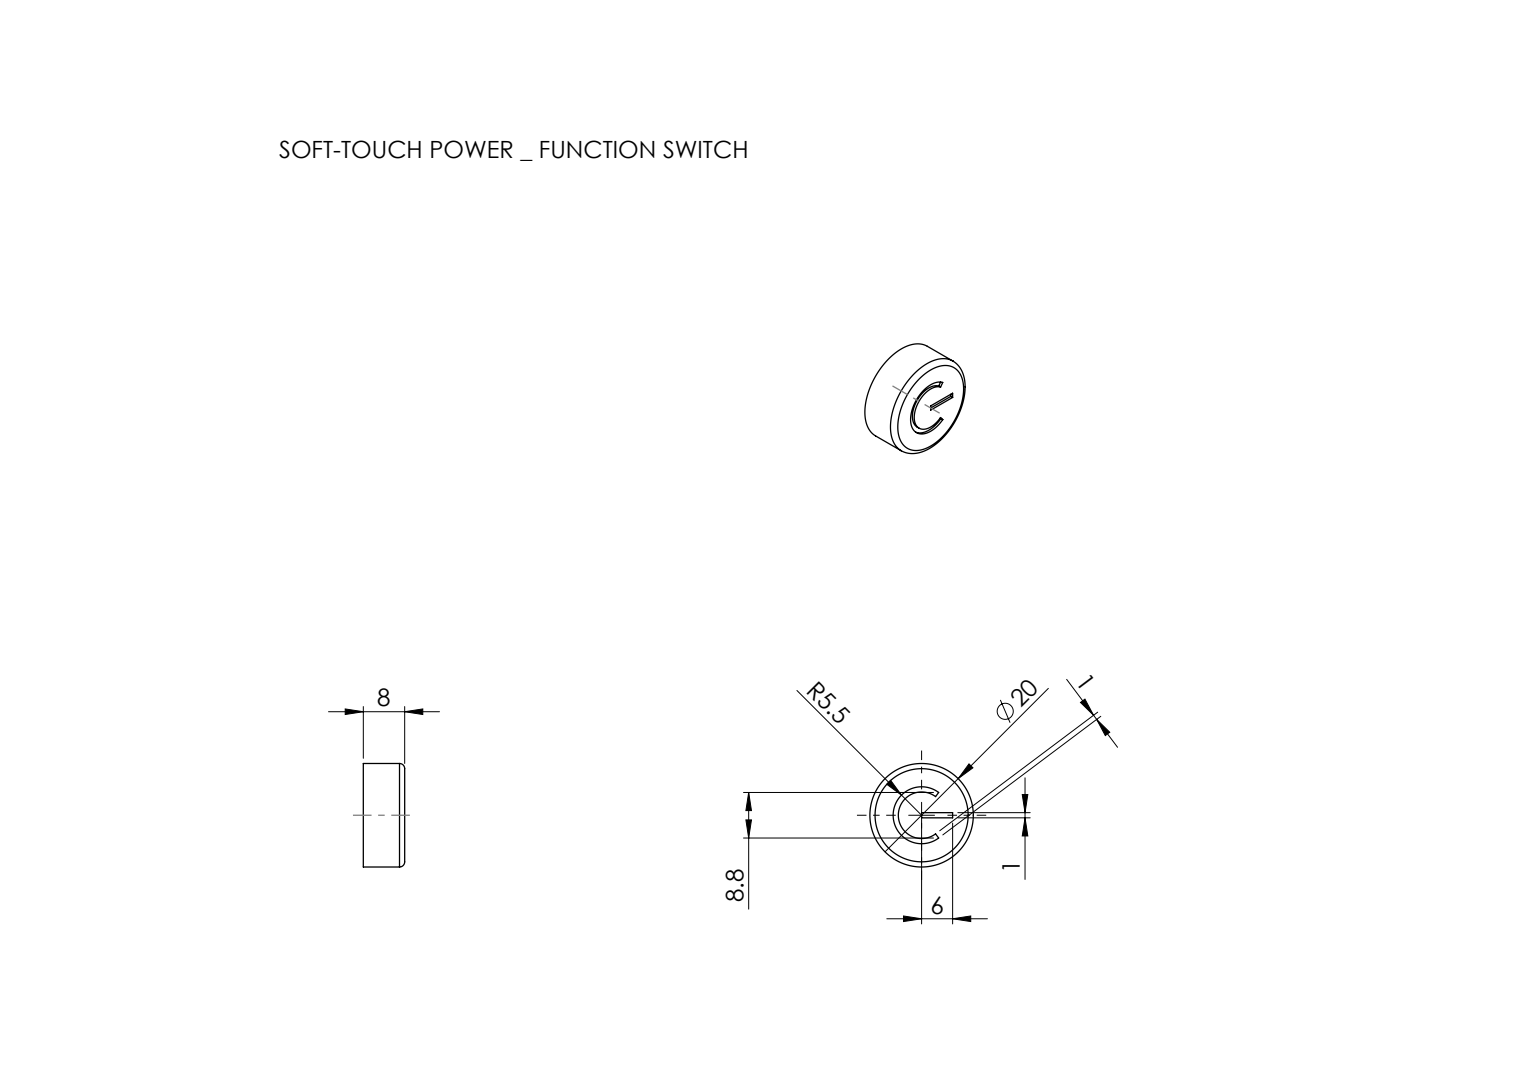
ISO-10303-21;
HEADER;
FILE_DESCRIPTION (('STEP AP214'),
    '1' );
FILE_NAME ('Soft-Touch Power _ Function Switch.step',
    '2026-10-08T15:02:10',
    ( '' ),
    ( '' ),
    'SwSTEP 2.0',
    'SolidWorks 2026',
    '' );
FILE_SCHEMA (( 'AUTOMOTIVE_DESIGN' ));
ENDSEC;

DATA;
#46=ORIENTED_EDGE ( 'NONE', *, *, #19993, .F. ) ;
#61=AXIS2_PLACEMENT_3D ( 'NONE', #8300, #8190, #21897 ) ;
#107=VECTOR ( 'NONE', #10777, 1000.000000000000000 ) ;
#129=CARTESIAN_POINT ( 'NONE',  ( 26.00000000000000000, -0.5000000000000000000, 0.000000000000000000 ) ) ;
#137=VERTEX_POINT ( 'NONE', #405 ) ;
#175=CARTESIAN_POINT ( 'NONE',  ( 26.00000000000000000, 0.5000000000000000000, 0.000000000000000000 ) ) ;
#230=DIRECTION ( 'NONE',  ( 0.000000000000000000, -1.000000000000000000, 0.000000000000000000 ) ) ;
#276=ORIENTED_EDGE ( 'NONE', *, *, #16709, .F. ) ;
#314=PRESENTATION_STYLE_ASSIGNMENT (( #17535 ) ) ;
#328=ORIENTED_EDGE ( 'NONE', *, *, #15715, .F. ) ;
#330=DIRECTION ( 'NONE',  ( 1.000000000000000000, 0.000000000000000000, 0.000000000000000000 ) ) ;
#379=FACE_OUTER_BOUND ( 'NONE', #20962, .T. ) ;
#386=EDGE_LOOP ( 'NONE', ( #10513, #13863, #2222, #14894 ) ) ;
#390=CARTESIAN_POINT ( 'NONE',  ( 25.50000000000000000, -0.5000000000000000000, 0.000000000000000000 ) ) ;
#405=CARTESIAN_POINT ( 'NONE',  ( 25.50000000000000000, -4.400000000000000355, -3.299999999999998490 ) ) ;
#408=DIRECTION ( 'NONE',  ( 1.000000000000000000, 0.000000000000000000, 0.000000000000000000 ) ) ;
#530=SURFACE_SIDE_STYLE ('',( #12575 ) ) ;
#566=VERTEX_POINT ( 'NONE', #2846 ) ;
#664=DIRECTION ( 'NONE',  ( 0.000000000000000000, 0.000000000000000000, -1.000000000000000000 ) ) ;
#679=AXIS2_PLACEMENT_3D ( 'NONE', #6039, #12809, #19760 ) ;
#731=CARTESIAN_POINT ( 'NONE',  ( 25.50000000000000000, 0.5000000000000000000, 0.000000000000000000 ) ) ;
#746=ADVANCED_FACE ( 'NONE', ( #18285 ), #1172, .T. ) ;
#770=CARTESIAN_POINT ( 'NONE',  ( 26.00000000000000000, 1.371657349757716727E-13, 9.000000000000001776 ) ) ;
#777=ORIENTED_EDGE ( 'NONE', *, *, #1994, .F. ) ;
#858=CARTESIAN_POINT ( 'NONE',  ( 26.00000000000000000, -0.5000000000000000000, 0.000000000000000000 ) ) ;
#976=ORIENTED_EDGE ( 'NONE', *, *, #5207, .F. ) ;
#1068=ORIENTED_EDGE ( 'NONE', *, *, #14661, .F. ) ;
#1075=CARTESIAN_POINT ( 'NONE',  ( 24.99999999999999645, 1.360023205165816762E-13, 10.00000000000000000 ) ) ;
#1088=ORIENTED_EDGE ( 'NONE', *, *, #2868, .F. ) ;
#1172=PLANE ( 'NONE',  #9056 ) ;
#1223=AXIS2_PLACEMENT_3D ( 'NONE', #21571, #2886, #14628 ) ;
#1293=EDGE_LOOP ( 'NONE', ( #4845, #14996, #17881, #4341 ) ) ;
#1397=VECTOR ( 'NONE', #13022, 1000.000000000000000 ) ;
#1428=PLANE ( 'NONE',  #21312 ) ;
#1693=DIRECTION ( 'NONE',  ( -1.000000000000000000, -0.000000000000000000, -0.000000000000000000 ) ) ;
#1761=LINE ( 'NONE', #8635, #13730 ) ;
#1967=DIRECTION ( 'NONE',  ( 0.000000000000000000, 0.000000000000000000, -1.000000000000000000 ) ) ;
#1994=EDGE_CURVE ( 'NONE', #6655, #4083, #3238, .T. ) ;
#2005=CARTESIAN_POINT ( 'NONE',  ( 26.00000000000000000, 0.000000000000000000, 0.000000000000000000 ) ) ;
#2048=DIRECTION ( 'NONE',  ( 1.000000000000000000, -0.000000000000000000, -0.000000000000000000 ) ) ;
#2170=AXIS2_PLACEMENT_3D ( 'NONE', #8967, #408, #3883 ) ;
#2214=ORIENTED_EDGE ( 'NONE', *, *, #11959, .F. ) ;
#2222=ORIENTED_EDGE ( 'NONE', *, *, #12958, .T. ) ;
#2243=ORIENTED_EDGE ( 'NONE', *, *, #15304, .F. ) ;
#2273=VECTOR ( 'NONE', #17556, 1000.000000000000000 ) ;
#2275=CARTESIAN_POINT ( 'NONE',  ( 26.00000000000000000, -4.400000000000000355, -3.299999999999998934 ) ) ;
#2285=ORIENTED_EDGE ( 'NONE', *, *, #5420, .T. ) ;
#2293=CARTESIAN_POINT ( 'NONE',  ( 24.99999999999999645, 1.371045026358143178E-13, 9.000000000000001776 ) ) ;
#2298=ORIENTED_EDGE ( 'NONE', *, *, #5629, .F. ) ;
#2331=CIRCLE ( 'NONE', #18866, 9.000000000000001776 ) ;
#2426=DIRECTION ( 'NONE',  ( 1.000000000000000000, -0.000000000000000000, -0.000000000000000000 ) ) ;
#2448=DIRECTION ( 'NONE',  ( -1.000000000000000000, 0.000000000000000000, -0.000000000000000000 ) ) ;
#2510=DIRECTION ( 'NONE',  ( 0.000000000000000000, -1.000000000000000000, 0.000000000000000000 ) ) ;
#2548=LINE ( 'NONE', #18093, #1397 ) ;
#2555=FACE_OUTER_BOUND ( 'NONE', #14128, .T. ) ;
#2588=ORIENTED_EDGE ( 'NONE', *, *, #4728, .F. ) ;
#2656=ORIENTED_EDGE ( 'NONE', *, *, #14942, .F. ) ;
#2672=EDGE_CURVE ( 'NONE', #6212, #9522, #7164, .T. ) ;
#2707=DIRECTION ( 'NONE',  ( 1.000000000000000000, 0.000000000000000000, 0.000000000000000000 ) ) ;
#2782=ADVANCED_FACE ( 'NONE', ( #19982 ), #6262, .F. ) ;
#2846=CARTESIAN_POINT ( 'NONE',  ( 25.50000000000000000, 0.5000000000000000000, -6.000000000000000000 ) ) ;
#2868=EDGE_CURVE ( 'NONE', #6745, #4083, #2548, .T. ) ;
#2886=DIRECTION ( 'NONE',  ( -1.000000000000000000, -0.000000000000000000, -0.000000000000000000 ) ) ;
#2913=FACE_OUTER_BOUND ( 'NONE', #3821, .T. ) ;
#2958=AXIS2_PLACEMENT_3D ( 'NONE', #14735, #19446, #4033 ) ;
#2986=CARTESIAN_POINT ( 'NONE',  ( 26.00000000000000000, 1.360023205165816762E-13, 0.000000000000000000 ) ) ;
#2998=( LENGTH_UNIT ( ) NAMED_UNIT ( * ) SI_UNIT ( .MILLI., .METRE. ) );
#3082=ORIENTED_EDGE ( 'NONE', *, *, #8473, .T. ) ;
#3119=CARTESIAN_POINT ( 'NONE',  ( 18.00000000000000000, 1.372269673157290277E-13, -10.00000000000000000 ) ) ;
#3159=CYLINDRICAL_SURFACE ( 'NONE', #11262, 4.500000000000000888 ) ;
#3238=LINE ( 'NONE', #3467, #7997 ) ;
#3252=EDGE_CURVE ( 'NONE', #12810, #12003, #3901, .T. ) ;
#3274=EDGE_LOOP ( 'NONE', ( #3082, #777, #2298, #22194 ) ) ;
#3321=CARTESIAN_POINT ( 'NONE',  ( 26.00000000000000000, -3.600000000000001421, -2.699999999999999289 ) ) ;
#3351=AXIS2_PLACEMENT_3D ( 'NONE', #14118, #5542, #19272 ) ;
#3391=VERTEX_POINT ( 'NONE', #3321 ) ;
#3436=DIRECTION ( 'NONE',  ( -1.000000000000000000, -0.000000000000000000, -0.000000000000000000 ) ) ;
#3467=CARTESIAN_POINT ( 'NONE',  ( 25.50000000000000000, -0.5000000000000000000, -6.000000000000000000 ) ) ;
#3474=ADVANCED_FACE ( 'NONE', ( #12002 ), #15162, .T. ) ;
#3756=DIRECTION ( 'NONE',  ( 0.000000000000000000, 1.000000000000000000, -1.224646799147353207E-16 ) ) ;
#3821=EDGE_LOOP ( 'NONE', ( #17497, #17029, #20739, #5281 ) ) ;
#3883=DIRECTION ( 'NONE',  ( 0.000000000000000000, 0.000000000000000000, -1.000000000000000000 ) ) ;
#3897=FILL_AREA_STYLE_COLOUR ( '', #6324 ) ;
#3901=CIRCLE ( 'NONE', #17927, 10.00000000000000000 ) ;
#4011=ORIENTED_EDGE ( 'NONE', *, *, #12403, .T. ) ;
#4032=LINE ( 'NONE', #21029, #9543 ) ;
#4033=DIRECTION ( 'NONE',  ( 0.000000000000000000, 0.000000000000000000, -1.000000000000000000 ) ) ;
#4043=AXIS2_PLACEMENT_3D ( 'NONE', #13177, #18133, #21596 ) ;
#4083=VERTEX_POINT ( 'NONE', #12114 ) ;
#4109=AXIS2_PLACEMENT_3D ( 'NONE', #10961, #16243, #16035 ) ;
#4115=CARTESIAN_POINT ( 'NONE',  ( 25.50000000000000000, -3.600000000000001421, -2.699999999999999289 ) ) ;
#4132=AXIS2_PLACEMENT_3D ( 'NONE', #7100, #230, #17449 ) ;
#4218=ORIENTED_EDGE ( 'NONE', *, *, #14942, .T. ) ;
#4341=ORIENTED_EDGE ( 'NONE', *, *, #14266, .F. ) ;
#4546=PRODUCT_CONTEXT ( 'NONE', #7149, 'mechanical' ) ;
#4609=DIRECTION ( 'NONE',  ( 0.000000000000000000, -0.7999999999999997113, 0.6000000000000004219 ) ) ;
#4614=CARTESIAN_POINT ( 'NONE',  ( 25.50000000000000000, 0.000000000000000000, 0.000000000000000000 ) ) ;
#4682=PRODUCT_DEFINITION_CONTEXT ( 'detailed design', #12889, 'design' ) ;
#4693=LINE ( 'NONE', #175, #9110 ) ;
#4720=SHAPE_REPRESENTATION_RELATIONSHIP ( 'NONE' , 'NONE' ,  #9901, #5876 ) ;
#4728=EDGE_CURVE ( 'NONE', #10662, #7309, #14691, .T. ) ;
#4793=DIRECTION ( 'NONE',  ( 0.000000000000000000, 1.000000000000000000, 0.000000000000000000 ) ) ;
#4845=ORIENTED_EDGE ( 'NONE', *, *, #5629, .T. ) ;
#4908=LINE ( 'NONE', #15393, #12641 ) ;
#5047=VECTOR ( 'NONE', #12562, 1000.000000000000000 ) ;
#5067=ORIENTED_EDGE ( 'NONE', *, *, #21758, .T. ) ;
#5125=DIRECTION ( 'NONE',  ( 0.000000000000000000, 0.000000000000000000, -1.000000000000000000 ) ) ;
#5207=EDGE_CURVE ( 'NONE', #10297, #15308, #1761, .T. ) ;
#5218=DIRECTION ( 'NONE',  ( 0.000000000000000000, 1.000000000000000000, 0.000000000000000000 ) ) ;
#5251=DIRECTION ( 'NONE',  ( 1.000000000000000000, -0.000000000000000000, -0.000000000000000000 ) ) ;
#5281=ORIENTED_EDGE ( 'NONE', *, *, #11865, .T. ) ;
#5358=CARTESIAN_POINT ( 'NONE',  ( 25.50000000000000000, -3.600000000000001421, -2.699999999999999289 ) ) ;
#5406=ADVANCED_FACE ( 'NONE', ( #8529 ), #13700, .T. ) ;
#5420=EDGE_CURVE ( 'NONE', #3391, #9522, #4908, .T. ) ;
#5519=DIRECTION ( 'NONE',  ( 0.000000000000000000, 0.000000000000000000, 1.000000000000000000 ) ) ;
#5531=DIRECTION ( 'NONE',  ( 0.000000000000000000, 0.000000000000000000, -1.000000000000000000 ) ) ;
#5542=DIRECTION ( 'NONE',  ( 1.000000000000000000, 0.000000000000000000, 0.000000000000000000 ) ) ;
#5592=DIRECTION ( 'NONE',  ( 0.000000000000000000, -0.7999999999999999334, -0.5999999999999999778 ) ) ;
#5624=ORIENTED_EDGE ( 'NONE', *, *, #15873, .T. ) ;
#5626=ORIENTED_EDGE ( 'NONE', *, *, #11865, .F. ) ;
#5629=EDGE_CURVE ( 'NONE', #15933, #6655, #6832, .T. ) ;
#5683=CARTESIAN_POINT ( 'NONE',  ( 25.50000000000000000, -0.5000000000000000000, 0.000000000000000000 ) ) ;
#5684=AXIS2_PLACEMENT_3D ( 'NONE', #2986, #3436, #20194 ) ;
#5695=CARTESIAN_POINT ( 'NONE',  ( 26.00000000000000000, 0.5000000000000000000, -6.000000000000000000 ) ) ;
#5819=EDGE_LOOP ( 'NONE', ( #17403, #18927 ) ) ;
#5855=PLANE ( 'NONE',  #4043 ) ;
#5870=DIRECTION ( 'NONE',  ( 0.000000000000000000, -0.7999999999999997113, 0.6000000000000004219 ) ) ;
#5873=EDGE_CURVE ( 'NONE', #19507, #13805, #10857, .T. ) ;
#5876=ADVANCED_BREP_SHAPE_REPRESENTATION ( '', ( #6798, #6677 ), #16347 ) ;
#5979=EDGE_CURVE ( 'NONE', #15933, #10297, #7395, .T. ) ;
#6039=CARTESIAN_POINT ( 'NONE',  ( 25.50000000000000000, -0.5000000000000000000, 0.000000000000000000 ) ) ;
#6045=CARTESIAN_POINT ( 'NONE',  ( 25.50000000000000000, -0.5000000000000000000, 0.000000000000000000 ) ) ;
#6048=FILL_AREA_STYLE ('',( #13253 ) ) ;
#6055=DIRECTION ( 'NONE',  ( 1.000000000000000000, 0.000000000000000000, 0.000000000000000000 ) ) ;
#6096=ADVANCED_FACE ( 'NONE', ( #8051 ), #16161, .T. ) ;
#6104=ADVANCED_FACE ( 'NONE', ( #12781 ), #21530, .T. ) ;
#6120=CARTESIAN_POINT ( 'NONE',  ( 26.00000000000000000, 4.399999999999999467, -3.300000000000000266 ) ) ;
#6212=VERTEX_POINT ( 'NONE', #6120 ) ;
#6262=PLANE ( 'NONE',  #679 ) ;
#6269=FACE_BOUND ( 'NONE', #11468, .T. ) ;
#6272=( NAMED_UNIT ( * ) SI_UNIT ( $, .STERADIAN. ) SOLID_ANGLE_UNIT ( ) );
#6296=AXIS2_PLACEMENT_3D ( 'NONE', #11354, #6055, #13153 ) ;
#6303=FACE_OUTER_BOUND ( 'NONE', #5819, .T. ) ;
#6324=COLOUR_RGB ( '', 0.09019608, 0.27058824, 0.51372549) ;
#6428=PRODUCT_DEFINITION ( 'UNKNOWN', '', #10679, #4682 ) ;
#6436=ORIENTED_EDGE ( 'NONE', *, *, #20861, .T. ) ;
#6606=DIRECTION ( 'NONE',  ( 0.000000000000000000, 0.000000000000000000, -1.000000000000000000 ) ) ;
#6617=CARTESIAN_POINT ( 'NONE',  ( 25.50000000000000000, -0.5000000000000000000, -6.000000000000000000 ) ) ;
#6655=VERTEX_POINT ( 'NONE', #6617 ) ;
#6662=DIRECTION ( 'NONE',  ( 1.000000000000000000, -0.000000000000000000, -0.000000000000000000 ) ) ;
#6677=AXIS2_PLACEMENT_3D ( 'NONE', #18028, #16226, #2707 ) ;
#6717=DIRECTION ( 'NONE',  ( 1.000000000000000000, 0.000000000000000000, 0.000000000000000000 ) ) ;
#6745=VERTEX_POINT ( 'NONE', #5695 ) ;
#6775=CARTESIAN_POINT ( 'NONE',  ( 25.50000000000000000, 0.000000000000000000, 0.000000000000000000 ) ) ;
#6798=MANIFOLD_SOLID_BREP ( 'Cut-Extrude-Thin1', #21569 ) ;
#6832=LINE ( 'NONE', #20535, #21975 ) ;
#6893=ORIENTED_EDGE ( 'NONE', *, *, #5207, .T. ) ;
#6953=AXIS2_PLACEMENT_3D ( 'NONE', #2293, #3756, #10641 ) ;
#6969=VERTEX_POINT ( 'NONE', #1075 ) ;
#6991=ORIENTED_EDGE ( 'NONE', *, *, #19993, .T. ) ;
#7022=CARTESIAN_POINT ( 'NONE',  ( 26.00000000000000000, 0.000000000000000000, 0.000000000000000000 ) ) ;
#7073=LINE ( 'NONE', #14167, #11264 ) ;
#7079=ORIENTED_EDGE ( 'NONE', *, *, #5873, .F. ) ;
#7100=CARTESIAN_POINT ( 'NONE',  ( 24.99999999999999645, 1.360023205165816762E-13, -9.000000000000001776 ) ) ;
#7149=APPLICATION_CONTEXT ( 'automotive_design' ) ;
#7164=CIRCLE ( 'NONE', #19005, 5.500000000000000000 ) ;
#7167=ORIENTED_EDGE ( 'NONE', *, *, #15545, .T. ) ;
#7198=DIRECTION ( 'NONE',  ( 0.000000000000000000, 0.000000000000000000, -1.000000000000000000 ) ) ;
#7227=CARTESIAN_POINT ( 'NONE',  ( 25.50000000000000000, 0.000000000000000000, 0.000000000000000000 ) ) ;
#7238=CARTESIAN_POINT ( 'NONE',  ( 26.00000000000000000, 3.600000000000000533, -2.700000000000000622 ) ) ;
#7269=ADVANCED_FACE ( 'NONE', ( #10493 ), #13884, .F. ) ;
#7309=VERTEX_POINT ( 'NONE', #7238 ) ;
#7322=CARTESIAN_POINT ( 'NONE',  ( 25.50000000000000000, 0.000000000000000000, 0.000000000000000000 ) ) ;
#7395=LINE ( 'NONE', #5683, #5047 ) ;
#7430=LINE ( 'NONE', #10692, #2273 ) ;
#7468=PLANE ( 'NONE',  #3351 ) ;
#7482=PLANE ( 'NONE',  #4109 ) ;
#7488=CARTESIAN_POINT ( 'NONE',  ( 25.50000000000000000, 0.5000000000000000000, -6.000000000000000000 ) ) ;
#7492=ORIENTED_EDGE ( 'NONE', *, *, #20798, .F. ) ;
#7619=( LENGTH_UNIT ( ) NAMED_UNIT ( * ) SI_UNIT ( .MILLI., .METRE. ) );
#7645=CARTESIAN_POINT ( 'NONE',  ( 18.00000000000000000, 1.360023205165816762E-13, 10.00000000000000000 ) ) ;
#7761=FACE_OUTER_BOUND ( 'NONE', #8438, .T. ) ;
#7865=SURFACE_STYLE_FILL_AREA ( #6048 ) ;
#7869=CARTESIAN_POINT ( 'NONE',  ( 25.50000000000000000, -3.600000000000001421, -2.699999999999999289 ) ) ;
#7970=SURFACE_SIDE_STYLE ('',( #7865 ) ) ;
#7997=VECTOR ( 'NONE', #10345, 1000.000000000000000 ) ;
#8008=CIRCLE ( 'NONE', #10527, 4.500000000000000888 ) ;
#8013=( NAMED_UNIT ( * ) SI_UNIT ( $, .STERADIAN. ) SOLID_ANGLE_UNIT ( ) );
#8051=FACE_OUTER_BOUND ( 'NONE', #386, .T. ) ;
#8084=CARTESIAN_POINT ( 'NONE',  ( 26.00000000000000000, 1.360023205165816762E-13, 0.000000000000000000 ) ) ;
#8102=ORIENTED_EDGE ( 'NONE', *, *, #12403, .F. ) ;
#8137=EDGE_CURVE ( 'NONE', #10662, #12137, #12816, .T. ) ;
#8190=DIRECTION ( 'NONE',  ( 0.000000000000000000, 0.000000000000000000, 1.000000000000000000 ) ) ;
#8197=( LENGTH_UNIT ( ) NAMED_UNIT ( * ) SI_UNIT ( .MILLI., .METRE. ) );
#8251=ORIENTED_EDGE ( 'NONE', *, *, #5979, .F. ) ;
#8300=CARTESIAN_POINT ( 'NONE',  ( 25.50000000000000000, 0.5000000000000000000, -6.000000000000000000 ) ) ;
#8373=DIRECTION ( 'NONE',  ( -1.000000000000000000, -0.000000000000000000, -0.000000000000000000 ) ) ;
#8384=CIRCLE ( 'NONE', #13780, 10.00000000000000000 ) ;
#8438=EDGE_LOOP ( 'NONE', ( #46, #9710, #2656, #15221 ) ) ;
#8473=EDGE_CURVE ( 'NONE', #10297, #4083, #19645, .T. ) ;
#8507=ORIENTED_EDGE ( 'NONE', *, *, #21758, .F. ) ;
#8529=FACE_OUTER_BOUND ( 'NONE', #17309, .T. ) ;
#8616=LINE ( 'NONE', #390, #18148 ) ;
#8635=CARTESIAN_POINT ( 'NONE',  ( 26.00000000000000000, -0.5000000000000000000, 0.000000000000000000 ) ) ;
#8870=DIRECTION ( 'NONE',  ( 0.000000000000000000, 0.000000000000000000, -1.000000000000000000 ) ) ;
#8914=DIRECTION ( 'NONE',  ( -1.000000000000000000, 0.000000000000000000, 0.000000000000000000 ) ) ;
#8967=CARTESIAN_POINT ( 'NONE',  ( 26.00000000000000000, 1.360023205165816762E-13, 0.000000000000000000 ) ) ;
#9051=EDGE_LOOP ( 'NONE', ( #6991, #21546, #11916, #8507 ) ) ;
#9056=AXIS2_PLACEMENT_3D ( 'NONE', #18392, #19733, #14915 ) ;
#9110=VECTOR ( 'NONE', #18442, 1000.000000000000000 ) ;
#9113=CARTESIAN_POINT ( 'NONE',  ( 25.50000000000000000, -4.400000000000000355, -3.299999999999998490 ) ) ;
#9171=CARTESIAN_POINT ( 'NONE',  ( 25.50000000000000000, 4.399999999999999467, -3.300000000000000266 ) ) ;
#9192=CIRCLE ( 'NONE', #21025, 5.500000000000000000 ) ;
#9202=EDGE_CURVE ( 'NONE', #7309, #3391, #8008, .T. ) ;
#9290=ORIENTED_EDGE ( 'NONE', *, *, #2672, .F. ) ;
#9402=DIRECTION ( 'NONE',  ( 0.000000000000000000, -1.000000000000000000, -0.000000000000000000 ) ) ;
#9433=ORIENTED_EDGE ( 'NONE', *, *, #8137, .T. ) ;
#9494=EDGE_CURVE ( 'NONE', #6212, #7309, #16233, .T. ) ;
#9516=DIRECTION ( 'NONE',  ( 0.000000000000000000, 0.000000000000000000, -1.000000000000000000 ) ) ;
#9522=VERTEX_POINT ( 'NONE', #2275 ) ;
#9525=COLOUR_RGB ( '', 0.09019608, 0.27058824, 0.51372549) ;
#9543=VECTOR ( 'NONE', #15764, 1000.000000000000000 ) ;
#9551=ADVANCED_FACE ( 'NONE', ( #379 ), #7468, .T. ) ;
#9629=EDGE_LOOP ( 'NONE', ( #17769, #6893, #20968, #17542 ) ) ;
#9710=ORIENTED_EDGE ( 'NONE', *, *, #20798, .T. ) ;
#9766=VECTOR ( 'NONE', #11305, 1000.000000000000000 ) ;
#9893=MECHANICAL_DESIGN_GEOMETRIC_PRESENTATION_REPRESENTATION('',(#22095),#19925);
#9901=SHAPE_REPRESENTATION ( 'Soft-Touch Power _ Function Switch', ( #6677 ), #16347 ) ;
#10003=CARTESIAN_POINT ( 'NONE',  ( 24.99999999999999645, 1.360023205165816762E-13, 0.000000000000000000 ) ) ;
#10026=LINE ( 'NONE', #15098, #20672 ) ;
#10135=DIRECTION ( 'NONE',  ( 0.000000000000000000, 0.000000000000000000, -1.000000000000000000 ) ) ;
#10168=CARTESIAN_POINT ( 'NONE',  ( 26.00000000000000000, 1.360023205165816762E-13, 10.00000000000000000 ) ) ;
#10205=EDGE_LOOP ( 'NONE', ( #18675, #2588, #9433, #11530 ) ) ;
#10265=CIRCLE ( 'NONE', #4132, 1.000000000000000888 ) ;
#10297=VERTEX_POINT ( 'NONE', #129 ) ;
#10345=DIRECTION ( 'NONE',  ( 1.000000000000000000, -0.000000000000000000, -0.000000000000000000 ) ) ;
#10493=FACE_OUTER_BOUND ( 'NONE', #15989, .T. ) ;
#10494=ADVANCED_FACE ( 'NONE', ( #11728 ), #3159, .T. ) ;
#10513=ORIENTED_EDGE ( 'NONE', *, *, #20477, .F. ) ;
#10527=AXIS2_PLACEMENT_3D ( 'NONE', #7022, #13894, #20731 ) ;
#10623=ADVANCED_FACE ( 'NONE', ( #21563 ), #14622, .F. ) ;
#10641=DIRECTION ( 'NONE',  ( 0.000000000000000000, 1.224646799147472769E-16, 1.000000000000000000 ) ) ;
#10662=VERTEX_POINT ( 'NONE', #11343 ) ;
#10679=PRODUCT_DEFINITION_FORMATION_WITH_SPECIFIED_SOURCE ( 'ANY', '', #13558, .NOT_KNOWN. ) ;
#10692=CARTESIAN_POINT ( 'NONE',  ( 25.50000000000000000, 0.5000000000000000000, -6.000000000000000000 ) ) ;
#10704=ORIENTED_EDGE ( 'NONE', *, *, #9494, .F. ) ;
#10731=CARTESIAN_POINT ( 'NONE',  ( 26.00000000000000000, 4.399999999999999467, -3.300000000000000266 ) ) ;
#10777=DIRECTION ( 'NONE',  ( 0.000000000000000000, 0.000000000000000000, -1.000000000000000000 ) ) ;
#10793=ADVANCED_FACE ( 'NONE', ( #2555 ), #16298, .T. ) ;
#10815=AXIS2_PLACEMENT_3D ( 'NONE', #731, #9402, #9516 ) ;
#10857=CIRCLE ( 'NONE', #2170, 9.000000000000001776 ) ;
#10879=FILL_AREA_STYLE ('',( #3897 ) ) ;
#10905=LINE ( 'NONE', #9113, #18463 ) ;
#10961=CARTESIAN_POINT ( 'NONE',  ( 25.50000000000000000, -3.600000000000001421, -2.699999999999999289 ) ) ;
#10997=( NAMED_UNIT ( * ) PLANE_ANGLE_UNIT ( ) SI_UNIT ( $, .RADIAN. ) );
#11048=EDGE_LOOP ( 'NONE', ( #7492, #8102, #5624, #7079 ) ) ;
#11079=LINE ( 'NONE', #7488, #15215 ) ;
#11128=CARTESIAN_POINT ( 'NONE',  ( 25.50000000000000000, 0.5000000000000000000, 0.000000000000000000 ) ) ;
#11262=AXIS2_PLACEMENT_3D ( 'NONE', #6775, #6662, #11949 ) ;
#11264=VECTOR ( 'NONE', #5251, 1000.000000000000000 ) ;
#11305=DIRECTION ( 'NONE',  ( 1.000000000000000000, -0.000000000000000000, -0.000000000000000000 ) ) ;
#11307=ADVANCED_FACE ( 'NONE', ( #6269, #16626, #19988 ), #1428, .T. ) ;
#11343=CARTESIAN_POINT ( 'NONE',  ( 25.50000000000000000, 3.600000000000000533, -2.700000000000000622 ) ) ;
#11354=CARTESIAN_POINT ( 'NONE',  ( 24.99999999999999645, 1.360023205165816762E-13, 0.000000000000000000 ) ) ;
#11468=EDGE_LOOP ( 'NONE', ( #9290, #15701, #19332, #2285 ) ) ;
#11491=CARTESIAN_POINT ( 'NONE',  ( 24.99999999999999645, 1.372269673157290277E-13, -10.00000000000000000 ) ) ;
#11530=ORIENTED_EDGE ( 'NONE', *, *, #13312, .T. ) ;
#11575=ORIENTED_EDGE ( 'NONE', *, *, #2672, .T. ) ;
#11599=CIRCLE ( 'NONE', #13053, 10.00000000000000000 ) ;
#11613=VECTOR ( 'NONE', #5592, 1000.000000000000227 ) ;
#11644=ORIENTED_EDGE ( 'NONE', *, *, #1994, .T. ) ;
#11728=FACE_OUTER_BOUND ( 'NONE', #10205, .T. ) ;
#11865=EDGE_CURVE ( 'NONE', #137, #9522, #10905, .T. ) ;
#11916=ORIENTED_EDGE ( 'NONE', *, *, #3252, .T. ) ;
#11949=DIRECTION ( 'NONE',  ( 0.000000000000000000, 0.000000000000000000, -1.000000000000000000 ) ) ;
#11959=EDGE_CURVE ( 'NONE', #566, #6745, #7430, .T. ) ;
#11973=TOROIDAL_SURFACE ( 'NONE', #2958, 9.000000000000001776, 1.000000000000000000 ) ;
#12002=FACE_OUTER_BOUND ( 'NONE', #9051, .T. ) ;
#12003=VERTEX_POINT ( 'NONE', #7645 ) ;
#12076=( GEOMETRIC_REPRESENTATION_CONTEXT ( 3 ) GLOBAL_UNCERTAINTY_ASSIGNED_CONTEXT ( ( #19550 ) ) GLOBAL_UNIT_ASSIGNED_CONTEXT ( ( #7619, #10997, #14050 ) ) REPRESENTATION_CONTEXT ( 'NONE', 'WORKASPACE' ) );
#12114=CARTESIAN_POINT ( 'NONE',  ( 26.00000000000000000, -0.5000000000000000000, -6.000000000000000000 ) ) ;
#12137=VERTEX_POINT ( 'NONE', #7869 ) ;
#12214=DIRECTION ( 'NONE',  ( 1.000000000000000000, 0.000000000000000000, 0.000000000000000000 ) ) ;
#12264=CARTESIAN_POINT ( 'NONE',  ( 25.50000000000000000, -0.5000000000000000000, 0.000000000000000000 ) ) ;
#12319=ORIENTED_EDGE ( 'NONE', *, *, #14661, .T. ) ;
#12363=ORIENTED_EDGE ( 'NONE', *, *, #20036, .T. ) ;
#12371=VERTEX_POINT ( 'NONE', #11128 ) ;
#12381=CARTESIAN_POINT ( 'NONE',  ( 25.50000000000000000, 4.399999999999999467, -3.300000000000000266 ) ) ;
#12403=EDGE_CURVE ( 'NONE', #22262, #6969, #17043, .T. ) ;
#12542=CARTESIAN_POINT ( 'NONE',  ( 26.00000000000000000, 1.360023205165816762E-13, 0.000000000000000000 ) ) ;
#12562=DIRECTION ( 'NONE',  ( 1.000000000000000000, -0.000000000000000000, -0.000000000000000000 ) ) ;
#12575=SURFACE_STYLE_FILL_AREA ( #10879 ) ;
#12608=ORIENTED_EDGE ( 'NONE', *, *, #16711, .F. ) ;
#12641=VECTOR ( 'NONE', #20198, 1000.000000000000227 ) ;
#12734=VECTOR ( 'NONE', #8870, 1000.000000000000000 ) ;
#12781=FACE_OUTER_BOUND ( 'NONE', #20760, .T. ) ;
#12802=MECHANICAL_DESIGN_GEOMETRIC_PRESENTATION_REPRESENTATION('',(#20325),#12076);
#12809=DIRECTION ( 'NONE',  ( 0.000000000000000000, -1.000000000000000000, -0.000000000000000000 ) ) ;
#12810=VERTEX_POINT ( 'NONE', #3119 ) ;
#12816=CIRCLE ( 'NONE', #13540, 4.500000000000000888 ) ;
#12889=APPLICATION_CONTEXT ( 'automotive_design' ) ;
#12958=EDGE_CURVE ( 'NONE', #12371, #566, #15068, .T. ) ;
#13022=DIRECTION ( 'NONE',  ( 0.000000000000000000, -1.000000000000000000, 0.000000000000000000 ) ) ;
#13053=AXIS2_PLACEMENT_3D ( 'NONE', #10003, #18330, #20751 ) ;
#13153=DIRECTION ( 'NONE',  ( 0.000000000000000000, 0.000000000000000000, -1.000000000000000000 ) ) ;
#13177=CARTESIAN_POINT ( 'NONE',  ( 18.00000000000000000, 1.360023205165816762E-13, 0.000000000000000000 ) ) ;
#13253=FILL_AREA_STYLE_COLOUR ( '', #9525 ) ;
#13312=EDGE_CURVE ( 'NONE', #12137, #3391, #19529, .T. ) ;
#13525=ORIENTED_EDGE ( 'NONE', *, *, #14266, .T. ) ;
#13526=AXIS2_PLACEMENT_3D ( 'NONE', #15563, #2048, #5531 ) ;
#13540=AXIS2_PLACEMENT_3D ( 'NONE', #4614, #18356, #16784 ) ;
#13558=PRODUCT ( 'Soft-Touch Power _ Function Switch', 'Soft-Touch Power _ Function Switch', '', ( #4546 ) ) ;
#13582=EDGE_LOOP ( 'NONE', ( #4218, #14367 ) ) ;
#13694=AXIS2_PLACEMENT_3D ( 'NONE', #19841, #19630, #16376 ) ;
#13700=PLANE ( 'NONE',  #61 ) ;
#13730=VECTOR ( 'NONE', #4793, 1000.000000000000000 ) ;
#13780=AXIS2_PLACEMENT_3D ( 'NONE', #20214, #12214, #1967 ) ;
#13805=VERTEX_POINT ( 'NONE', #14928 ) ;
#13863=ORIENTED_EDGE ( 'NONE', *, *, #15545, .F. ) ;
#13884=CYLINDRICAL_SURFACE ( 'NONE', #13526, 5.500000000000000000 ) ;
#13894=DIRECTION ( 'NONE',  ( 1.000000000000000000, 0.000000000000000000, 0.000000000000000000 ) ) ;
#14033=EDGE_LOOP ( 'NONE', ( #10704, #276, #12319, #15281 ) ) ;
#14050=( NAMED_UNIT ( * ) SI_UNIT ( $, .STERADIAN. ) SOLID_ANGLE_UNIT ( ) );
#14118=CARTESIAN_POINT ( 'NONE',  ( 25.50000000000000000, 0.000000000000000000, 0.000000000000000000 ) ) ;
#14128=EDGE_LOOP ( 'NONE', ( #976, #8251, #13525, #7167 ) ) ;
#14157=AXIS2_PLACEMENT_3D ( 'NONE', #6045, #18099, #2448 ) ;
#14167=CARTESIAN_POINT ( 'NONE',  ( 25.50000000000000000, 4.399999999999999467, -3.300000000000000266 ) ) ;
#14191=DIRECTION ( 'NONE',  ( 1.000000000000000000, 0.000000000000000000, 0.000000000000000000 ) ) ;
#14266=EDGE_CURVE ( 'NONE', #15933, #12371, #8616, .T. ) ;
#14367=ORIENTED_EDGE ( 'NONE', *, *, #5873, .T. ) ;
#14541=VECTOR ( 'NONE', #2426, 1000.000000000000000 ) ;
#14589=ADVANCED_FACE ( 'NONE', ( #2913 ), #7482, .T. ) ;
#14622=PLANE ( 'NONE',  #18451 ) ;
#14628=DIRECTION ( 'NONE',  ( 0.000000000000000000, 0.000000000000000000, -1.000000000000000000 ) ) ;
#14661=EDGE_CURVE ( 'NONE', #15877, #10662, #14984, .T. ) ;
#14691=LINE ( 'NONE', #19836, #9766 ) ;
#14735=CARTESIAN_POINT ( 'NONE',  ( 24.99999999999999645, 1.360023205165816762E-13, 0.000000000000000000 ) ) ;
#14894=ORIENTED_EDGE ( 'NONE', *, *, #11959, .T. ) ;
#14915=DIRECTION ( 'NONE',  ( 0.000000000000000000, -0.7999999999999997113, 0.6000000000000004219 ) ) ;
#14928=CARTESIAN_POINT ( 'NONE',  ( 26.00000000000000000, 1.360023205165816762E-13, -9.000000000000001776 ) ) ;
#14942=EDGE_CURVE ( 'NONE', #13805, #19507, #2331, .T. ) ;
#14984=LINE ( 'NONE', #9171, #15635 ) ;
#14996=ORIENTED_EDGE ( 'NONE', *, *, #20861, .F. ) ;
#15068=LINE ( 'NONE', #19315, #12734 ) ;
#15098=CARTESIAN_POINT ( 'NONE',  ( 26.00000000000000000, 1.372269673157290277E-13, -10.00000000000000000 ) ) ;
#15162=CYLINDRICAL_SURFACE ( 'NONE', #5684, 10.00000000000000000 ) ;
#15215=VECTOR ( 'NONE', #2510, 1000.000000000000000 ) ;
#15221=ORIENTED_EDGE ( 'NONE', *, *, #15873, .F. ) ;
#15281=ORIENTED_EDGE ( 'NONE', *, *, #4728, .T. ) ;
#15304=EDGE_CURVE ( 'NONE', #22262, #12810, #10026, .T. ) ;
#15308=VERTEX_POINT ( 'NONE', #17220 ) ;
#15362=PRODUCT_DEFINITION_SHAPE ( 'NONE', 'NONE',  #6428 ) ;
#15393=CARTESIAN_POINT ( 'NONE',  ( 26.00000000000000000, -3.600000000000001421, -2.699999999999999289 ) ) ;
#15545=EDGE_CURVE ( 'NONE', #12371, #15308, #4032, .T. ) ;
#15563=CARTESIAN_POINT ( 'NONE',  ( 25.50000000000000000, 0.000000000000000000, 0.000000000000000000 ) ) ;
#15586=ORIENTED_EDGE ( 'NONE', *, *, #16709, .T. ) ;
#15635=VECTOR ( 'NONE', #4609, 999.9999999999998863 ) ;
#15701=ORIENTED_EDGE ( 'NONE', *, *, #9494, .T. ) ;
#15715=EDGE_CURVE ( 'NONE', #15877, #137, #9192, .T. ) ;
#15764=DIRECTION ( 'NONE',  ( 1.000000000000000000, -0.000000000000000000, -0.000000000000000000 ) ) ;
#15873=EDGE_CURVE ( 'NONE', #22262, #13805, #10265, .T. ) ;
#15877=VERTEX_POINT ( 'NONE', #12381 ) ;
#15933=VERTEX_POINT ( 'NONE', #12264 ) ;
#15989=EDGE_LOOP ( 'NONE', ( #11575, #5626, #328, #15586 ) ) ;
#16035=DIRECTION ( 'NONE',  ( 0.000000000000000000, -0.7999999999999999334, -0.6000000000000000888 ) ) ;
#16161=PLANE ( 'NONE',  #10815 ) ;
#16226=DIRECTION ( 'NONE',  ( 0.000000000000000000, 0.000000000000000000, 1.000000000000000000 ) ) ;
#16233=LINE ( 'NONE', #10731, #18077 ) ;
#16243=DIRECTION ( 'NONE',  ( 0.000000000000000000, -0.6000000000000000888, 0.7999999999999999334 ) ) ;
#16298=PLANE ( 'NONE',  #14157 ) ;
#16347=( GEOMETRIC_REPRESENTATION_CONTEXT ( 3 ) GLOBAL_UNCERTAINTY_ASSIGNED_CONTEXT ( ( #21128 ) ) GLOBAL_UNIT_ASSIGNED_CONTEXT ( ( #8197, #18217, #6272 ) ) REPRESENTATION_CONTEXT ( 'NONE', 'WORKASPACE' ) );
#16376=DIRECTION ( 'NONE',  ( 0.000000000000000000, 0.000000000000000000, 1.000000000000000000 ) ) ;
#16390=ADVANCED_FACE ( 'NONE', ( #7761 ), #18514, .T. ) ;
#16510=CARTESIAN_POINT ( 'NONE',  ( 18.00000000000000000, 1.360023205165816762E-13, 0.000000000000000000 ) ) ;
#16626=FACE_BOUND ( 'NONE', #9629, .T. ) ;
#16650=CIRCLE ( 'NONE', #6953, 1.000000000000000888 ) ;
#16709=EDGE_CURVE ( 'NONE', #15877, #6212, #7073, .T. ) ;
#16711=EDGE_CURVE ( 'NONE', #12137, #137, #17642, .T. ) ;
#16784=DIRECTION ( 'NONE',  ( 0.000000000000000000, 0.000000000000000000, -1.000000000000000000 ) ) ;
#16852=DIRECTION ( 'NONE',  ( 1.000000000000000000, 0.000000000000000000, 0.000000000000000000 ) ) ;
#16888=DIRECTION ( 'NONE',  ( 1.000000000000000000, 0.000000000000000000, 0.000000000000000000 ) ) ;
#17029=ORIENTED_EDGE ( 'NONE', *, *, #13312, .F. ) ;
#17043=CIRCLE ( 'NONE', #1223, 10.00000000000000000 ) ;
#17180=DIRECTION ( 'NONE',  ( 0.000000000000000000, 0.000000000000000000, -1.000000000000000000 ) ) ;
#17220=CARTESIAN_POINT ( 'NONE',  ( 26.00000000000000000, 0.5000000000000000000, 0.000000000000000000 ) ) ;
#17309=EDGE_LOOP ( 'NONE', ( #1088, #2214, #6436, #11644 ) ) ;
#17403=ORIENTED_EDGE ( 'NONE', *, *, #20036, .F. ) ;
#17445=DIRECTION ( 'NONE',  ( 1.000000000000000000, -0.000000000000000000, -0.000000000000000000 ) ) ;
#17449=DIRECTION ( 'NONE',  ( 0.000000000000000000, 0.000000000000000000, -1.000000000000000000 ) ) ;
#17497=ORIENTED_EDGE ( 'NONE', *, *, #5420, .F. ) ;
#17535=SURFACE_STYLE_USAGE ( .BOTH. , #530 ) ;
#17542=ORIENTED_EDGE ( 'NONE', *, *, #2868, .T. ) ;
#17556=DIRECTION ( 'NONE',  ( 1.000000000000000000, -0.000000000000000000, -0.000000000000000000 ) ) ;
#17642=LINE ( 'NONE', #5358, #11613 ) ;
#17744=SHAPE_DEFINITION_REPRESENTATION ( #15362, #9901 ) ;
#17769=ORIENTED_EDGE ( 'NONE', *, *, #8473, .F. ) ;
#17881=ORIENTED_EDGE ( 'NONE', *, *, #12958, .F. ) ;
#17927=AXIS2_PLACEMENT_3D ( 'NONE', #16510, #6717, #17180 ) ;
#18028=CARTESIAN_POINT ( 'NONE',  ( 0.000000000000000000, 0.000000000000000000, 0.000000000000000000 ) ) ;
#18077=VECTOR ( 'NONE', #5870, 999.9999999999998863 ) ;
#18093=CARTESIAN_POINT ( 'NONE',  ( 26.00000000000000000, 0.5000000000000000000, -6.000000000000000000 ) ) ;
#18099=DIRECTION ( 'NONE',  ( 0.000000000000000000, 0.000000000000000000, -1.000000000000000000 ) ) ;
#18133=DIRECTION ( 'NONE',  ( 1.000000000000000000, 0.000000000000000000, 0.000000000000000000 ) ) ;
#18148=VECTOR ( 'NONE', #5218, 1000.000000000000000 ) ;
#18217=( NAMED_UNIT ( * ) PLANE_ANGLE_UNIT ( ) SI_UNIT ( $, .RADIAN. ) );
#18285=FACE_OUTER_BOUND ( 'NONE', #14033, .T. ) ;
#18330=DIRECTION ( 'NONE',  ( -1.000000000000000000, -0.000000000000000000, -0.000000000000000000 ) ) ;
#18356=DIRECTION ( 'NONE',  ( 1.000000000000000000, 0.000000000000000000, 0.000000000000000000 ) ) ;
#18379=ADVANCED_FACE ( 'NONE', ( #6303 ), #5855, .F. ) ;
#18392=CARTESIAN_POINT ( 'NONE',  ( 25.50000000000000000, 4.399999999999999467, -3.300000000000000266 ) ) ;
#18442=DIRECTION ( 'NONE',  ( 0.000000000000000000, 0.000000000000000000, -1.000000000000000000 ) ) ;
#18451=AXIS2_PLACEMENT_3D ( 'NONE', #7227, #8914, #5519 ) ;
#18463=VECTOR ( 'NONE', #17445, 1000.000000000000000 ) ;
#18514=TOROIDAL_SURFACE ( 'NONE', #6296, 9.000000000000001776, 1.000000000000000000 ) ;
#18675=ORIENTED_EDGE ( 'NONE', *, *, #9202, .F. ) ;
#18719=LINE ( 'NONE', #10168, #22112 ) ;
#18866=AXIS2_PLACEMENT_3D ( 'NONE', #12542, #16888, #10135 ) ;
#18927=ORIENTED_EDGE ( 'NONE', *, *, #3252, .F. ) ;
#19005=AXIS2_PLACEMENT_3D ( 'NONE', #2005, #330, #7198 ) ;
#19272=DIRECTION ( 'NONE',  ( 0.000000000000000000, 0.000000000000000000, -1.000000000000000000 ) ) ;
#19315=CARTESIAN_POINT ( 'NONE',  ( 25.50000000000000000, 0.5000000000000000000, 0.000000000000000000 ) ) ;
#19332=ORIENTED_EDGE ( 'NONE', *, *, #9202, .T. ) ;
#19446=DIRECTION ( 'NONE',  ( 1.000000000000000000, 0.000000000000000000, 0.000000000000000000 ) ) ;
#19507=VERTEX_POINT ( 'NONE', #770 ) ;
#19529=LINE ( 'NONE', #4115, #14541 ) ;
#19550=UNCERTAINTY_MEASURE_WITH_UNIT (LENGTH_MEASURE( 1.000000000000000082E-05 ), #7619, 'distance_accuracy_value', 'NONE');
#19630=DIRECTION ( 'NONE',  ( -1.000000000000000000, -0.000000000000000000, -0.000000000000000000 ) ) ;
#19645=LINE ( 'NONE', #858, #107 ) ;
#19733=DIRECTION ( 'NONE',  ( 0.000000000000000000, 0.6000000000000004219, 0.7999999999999997113 ) ) ;
#19760=DIRECTION ( 'NONE',  ( 0.000000000000000000, 0.000000000000000000, -1.000000000000000000 ) ) ;
#19769=PRESENTATION_STYLE_ASSIGNMENT (( #21795 ) ) ;
#19834=ADVANCED_FACE ( 'NONE', ( #21688 ), #11973, .T. ) ;
#19836=CARTESIAN_POINT ( 'NONE',  ( 25.50000000000000000, 3.600000000000000533, -2.700000000000000622 ) ) ;
#19841=CARTESIAN_POINT ( 'NONE',  ( 26.00000000000000000, 1.360023205165816762E-13, 0.000000000000000000 ) ) ;
#19925=( GEOMETRIC_REPRESENTATION_CONTEXT ( 3 ) GLOBAL_UNCERTAINTY_ASSIGNED_CONTEXT ( ( #22011 ) ) GLOBAL_UNIT_ASSIGNED_CONTEXT ( ( #2998, #21681, #8013 ) ) REPRESENTATION_CONTEXT ( 'NONE', 'WORKASPACE' ) );
#19982=FACE_OUTER_BOUND ( 'NONE', #3274, .T. ) ;
#19988=FACE_OUTER_BOUND ( 'NONE', #13582, .T. ) ;
#19993=EDGE_CURVE ( 'NONE', #6969, #22262, #11599, .T. ) ;
#20036=EDGE_CURVE ( 'NONE', #12003, #12810, #8384, .T. ) ;
#20194=DIRECTION ( 'NONE',  ( 0.000000000000000000, 0.000000000000000000, 1.000000000000000000 ) ) ;
#20198=DIRECTION ( 'NONE',  ( 0.000000000000000000, -0.7999999999999999334, -0.5999999999999999778 ) ) ;
#20214=CARTESIAN_POINT ( 'NONE',  ( 18.00000000000000000, 1.360023205165816762E-13, 0.000000000000000000 ) ) ;
#20325=STYLED_ITEM ( 'NONE', ( #314 ), #6798 ) ;
#20477=EDGE_CURVE ( 'NONE', #15308, #6745, #4693, .T. ) ;
#20535=CARTESIAN_POINT ( 'NONE',  ( 25.50000000000000000, -0.5000000000000000000, 0.000000000000000000 ) ) ;
#20672=VECTOR ( 'NONE', #1693, 1000.000000000000000 ) ;
#20731=DIRECTION ( 'NONE',  ( 0.000000000000000000, 0.000000000000000000, -1.000000000000000000 ) ) ;
#20739=ORIENTED_EDGE ( 'NONE', *, *, #16711, .T. ) ;
#20751=DIRECTION ( 'NONE',  ( 0.000000000000000000, 0.000000000000000000, -1.000000000000000000 ) ) ;
#20760=EDGE_LOOP ( 'NONE', ( #2243, #4011, #5067, #12363 ) ) ;
#20798=EDGE_CURVE ( 'NONE', #6969, #19507, #16650, .T. ) ;
#20861=EDGE_CURVE ( 'NONE', #566, #6655, #11079, .T. ) ;
#20962=EDGE_LOOP ( 'NONE', ( #21999, #12608, #21535, #1068 ) ) ;
#20968=ORIENTED_EDGE ( 'NONE', *, *, #20477, .T. ) ;
#21025=AXIS2_PLACEMENT_3D ( 'NONE', #7322, #14191, #664 ) ;
#21029=CARTESIAN_POINT ( 'NONE',  ( 25.50000000000000000, 0.5000000000000000000, 0.000000000000000000 ) ) ;
#21128=UNCERTAINTY_MEASURE_WITH_UNIT (LENGTH_MEASURE( 1.000000000000000082E-05 ), #8197, 'distance_accuracy_value', 'NONE');
#21312=AXIS2_PLACEMENT_3D ( 'NONE', #8084, #16852, #6606 ) ;
#21530=CYLINDRICAL_SURFACE ( 'NONE', #13694, 10.00000000000000000 ) ;
#21535=ORIENTED_EDGE ( 'NONE', *, *, #8137, .F. ) ;
#21546=ORIENTED_EDGE ( 'NONE', *, *, #15304, .T. ) ;
#21563=FACE_OUTER_BOUND ( 'NONE', #1293, .T. ) ;
#21569=CLOSED_SHELL ( 'NONE', ( #16390, #3474, #6104, #11307, #18379, #19834, #2782, #10793, #6096, #5406, #10623, #7269, #746, #10494, #14589, #9551 ) ) ;
#21571=CARTESIAN_POINT ( 'NONE',  ( 24.99999999999999645, 1.360023205165816762E-13, 0.000000000000000000 ) ) ;
#21596=DIRECTION ( 'NONE',  ( 0.000000000000000000, 0.000000000000000000, -1.000000000000000000 ) ) ;
#21681=( NAMED_UNIT ( * ) PLANE_ANGLE_UNIT ( ) SI_UNIT ( $, .RADIAN. ) );
#21688=FACE_OUTER_BOUND ( 'NONE', #11048, .T. ) ;
#21758=EDGE_CURVE ( 'NONE', #6969, #12003, #18719, .T. ) ;
#21795=SURFACE_STYLE_USAGE ( .BOTH. , #7970 ) ;
#21897=DIRECTION ( 'NONE',  ( 1.000000000000000000, 0.000000000000000000, -0.000000000000000000 ) ) ;
#21975=VECTOR ( 'NONE', #5125, 1000.000000000000000 ) ;
#21999=ORIENTED_EDGE ( 'NONE', *, *, #15715, .T. ) ;
#22011=UNCERTAINTY_MEASURE_WITH_UNIT (LENGTH_MEASURE( 1.000000000000000082E-05 ), #2998, 'distance_accuracy_value', 'NONE');
#22095=STYLED_ITEM ( 'NONE', ( #19769 ), #5876 ) ;
#22112=VECTOR ( 'NONE', #8373, 1000.000000000000000 ) ;
#22194=ORIENTED_EDGE ( 'NONE', *, *, #5979, .T. ) ;
#22262=VERTEX_POINT ( 'NONE', #11491 ) ;
ENDSEC;
END-ISO-10303-21;
